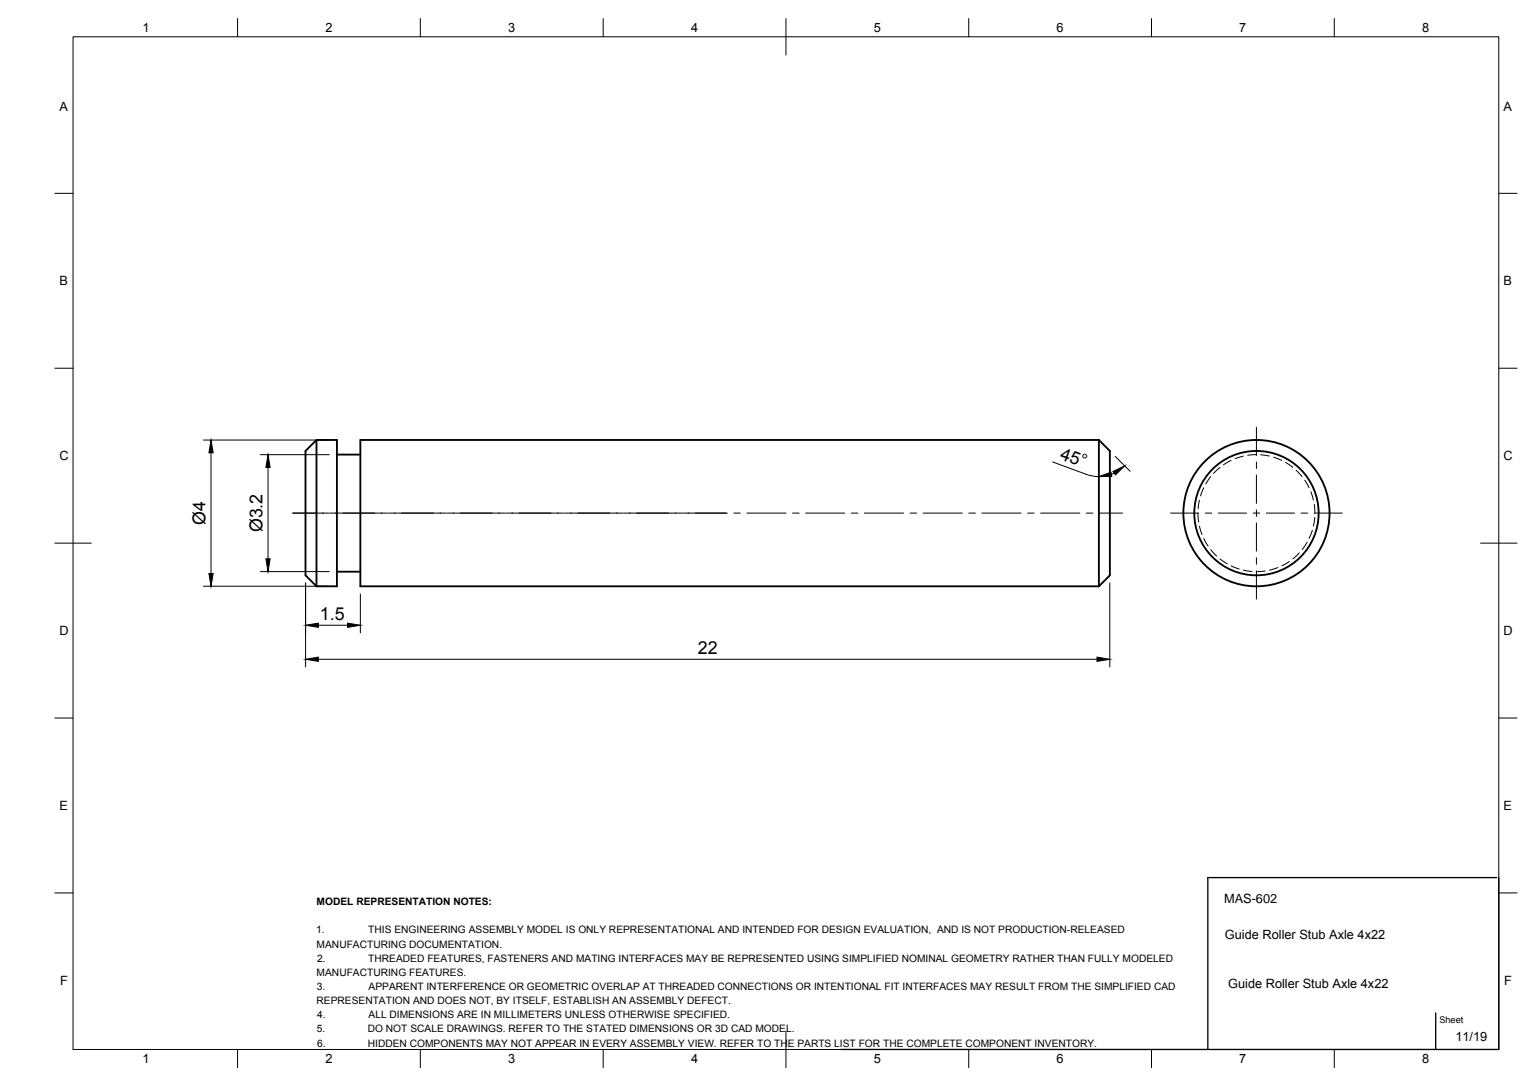
ISO-10303-21;
HEADER;
/* Generated by software containing ST-Developer
 * from STEP Tools, Inc. (www.steptools.com) 
 */

FILE_DESCRIPTION(
/* description */ (''),
/* implementation_level */ '2;1');

FILE_NAME(
/* name */ 'Guide Roller Stub Axle 4x22.step',
/* time_stamp */ '2026-10-15T14:42:47-07:00',
/* author */ (''),
/* organization */ (''),
/* preprocessor_version */ 'ST-DEVELOPER v20.2',
/* originating_system */ 'Autodesk Translation Framework v15.15.0.0',
/* authorisation */ '');

FILE_SCHEMA (('AUTOMOTIVE_DESIGN { 1 0 10303 214 3 1 1 }'));
ENDSEC;

DATA;
#10=MECHANICAL_DESIGN_GEOMETRIC_PRESENTATION_REPRESENTATION('',(#247),#85789);
#187=CONICAL_SURFACE('',#10762,0.185,0.78539816339745);
#188=CONICAL_SURFACE('',#10774,0.185,0.785398163397445);
#211=SHAPE_REPRESENTATION_RELATIONSHIP('SRR','None',#85876,#229);
#229=ADVANCED_BREP_SHAPE_REPRESENTATION('',(#265),#85784);
#247=STYLED_ITEM('',(#85975),#265);
#265=MANIFOLD_SOLID_BREP('Body1',#9894);
#471=FACE_BOUND('',#3409,.T.);
#472=FACE_BOUND('',#3412,.T.);
#1171=PLANE('',#10760);
#1172=PLANE('',#10766);
#1173=PLANE('',#10770);
#1174=PLANE('',#10776);
#1655=LINE('',#77849,#2191);
#1656=LINE('',#77853,#2192);
#1657=LINE('',#77860,#2193);
#1658=LINE('',#77867,#2194);
#1659=LINE('',#77870,#2195);
#2191=VECTOR('',#12747,0.185);
#2192=VECTOR('',#12752,0.2);
#2193=VECTOR('',#12761,0.16);
#2194=VECTOR('',#12770,0.2);
#2195=VECTOR('',#12773,0.185);
#2361=CYLINDRICAL_SURFACE('',#10764,0.2);
#2362=CYLINDRICAL_SURFACE('',#10768,0.16);
#2363=CYLINDRICAL_SURFACE('',#10772,0.2);
#2819=FACE_OUTER_BOUND('',#3405,.T.);
#2820=FACE_OUTER_BOUND('',#3406,.T.);
#2821=FACE_OUTER_BOUND('',#3407,.T.);
#2822=FACE_OUTER_BOUND('',#3408,.T.);
#2823=FACE_OUTER_BOUND('',#3410,.T.);
#2824=FACE_OUTER_BOUND('',#3411,.T.);
#2825=FACE_OUTER_BOUND('',#3413,.T.);
#2826=FACE_OUTER_BOUND('',#3414,.T.);
#2827=FACE_OUTER_BOUND('',#3415,.T.);
#3405=EDGE_LOOP('',(#8863));
#3406=EDGE_LOOP('',(#8864,#8865,#8866,#8867));
#3407=EDGE_LOOP('',(#8868,#8869,#8870,#8871));
#3408=EDGE_LOOP('',(#8872));
#3409=EDGE_LOOP('',(#8873));
#3410=EDGE_LOOP('',(#8874,#8875,#8876,#8877));
#3411=EDGE_LOOP('',(#8878));
#3412=EDGE_LOOP('',(#8879));
#3413=EDGE_LOOP('',(#8880,#8881,#8882,#8883));
#3414=EDGE_LOOP('',(#8884,#8885,#8886,#8887));
#3415=EDGE_LOOP('',(#8888));
#3812=CIRCLE('',#10761,0.17);
#3813=CIRCLE('',#10763,0.2);
#3814=CIRCLE('',#10765,0.2);
#3815=CIRCLE('',#10767,0.16);
#3816=CIRCLE('',#10769,0.16);
#3817=CIRCLE('',#10771,0.2);
#3818=CIRCLE('',#10773,0.2);
#3819=CIRCLE('',#10775,0.17);
#4749=VERTEX_POINT('',#77844);
#4750=VERTEX_POINT('',#77847);
#4751=VERTEX_POINT('',#77851);
#4752=VERTEX_POINT('',#77855);
#4753=VERTEX_POINT('',#77858);
#4754=VERTEX_POINT('',#77862);
#4755=VERTEX_POINT('',#77865);
#4756=VERTEX_POINT('',#77869);
#6159=EDGE_CURVE('',#4749,#4749,#3812,.T.);
#6160=EDGE_CURVE('',#4750,#4750,#3813,.T.);
#6161=EDGE_CURVE('',#4750,#4749,#1655,.T.);
#6162=EDGE_CURVE('',#4751,#4751,#3814,.T.);
#6163=EDGE_CURVE('',#4751,#4750,#1656,.T.);
#6164=EDGE_CURVE('',#4752,#4752,#3815,.T.);
#6165=EDGE_CURVE('',#4753,#4753,#3816,.T.);
#6166=EDGE_CURVE('',#4753,#4752,#1657,.T.);
#6167=EDGE_CURVE('',#4754,#4754,#3817,.T.);
#6168=EDGE_CURVE('',#4755,#4755,#3818,.T.);
#6169=EDGE_CURVE('',#4755,#4754,#1658,.T.);
#6170=EDGE_CURVE('',#4755,#4756,#1659,.T.);
#6171=EDGE_CURVE('',#4756,#4756,#3819,.T.);
#8863=ORIENTED_EDGE('',*,*,#6159,.F.);
#8864=ORIENTED_EDGE('',*,*,#6160,.F.);
#8865=ORIENTED_EDGE('',*,*,#6161,.T.);
#8866=ORIENTED_EDGE('',*,*,#6159,.T.);
#8867=ORIENTED_EDGE('',*,*,#6161,.F.);
#8868=ORIENTED_EDGE('',*,*,#6162,.F.);
#8869=ORIENTED_EDGE('',*,*,#6163,.T.);
#8870=ORIENTED_EDGE('',*,*,#6160,.T.);
#8871=ORIENTED_EDGE('',*,*,#6163,.F.);
#8872=ORIENTED_EDGE('',*,*,#6162,.T.);
#8873=ORIENTED_EDGE('',*,*,#6164,.F.);
#8874=ORIENTED_EDGE('',*,*,#6165,.F.);
#8875=ORIENTED_EDGE('',*,*,#6166,.T.);
#8876=ORIENTED_EDGE('',*,*,#6164,.T.);
#8877=ORIENTED_EDGE('',*,*,#6166,.F.);
#8878=ORIENTED_EDGE('',*,*,#6167,.F.);
#8879=ORIENTED_EDGE('',*,*,#6165,.T.);
#8880=ORIENTED_EDGE('',*,*,#6168,.F.);
#8881=ORIENTED_EDGE('',*,*,#6169,.T.);
#8882=ORIENTED_EDGE('',*,*,#6167,.T.);
#8883=ORIENTED_EDGE('',*,*,#6169,.F.);
#8884=ORIENTED_EDGE('',*,*,#6168,.T.);
#8885=ORIENTED_EDGE('',*,*,#6170,.T.);
#8886=ORIENTED_EDGE('',*,*,#6171,.F.);
#8887=ORIENTED_EDGE('',*,*,#6170,.F.);
#8888=ORIENTED_EDGE('',*,*,#6171,.T.);
#9797=ADVANCED_FACE('',(#2819),#1171,.T.);
#9798=ADVANCED_FACE('',(#2820),#187,.T.);
#9799=ADVANCED_FACE('',(#2821),#2361,.T.);
#9800=ADVANCED_FACE('',(#2822,#471),#1172,.T.);
#9801=ADVANCED_FACE('',(#2823),#2362,.T.);
#9802=ADVANCED_FACE('',(#2824,#472),#1173,.T.);
#9803=ADVANCED_FACE('',(#2825),#2363,.T.);
#9804=ADVANCED_FACE('',(#2826),#188,.T.);
#9805=ADVANCED_FACE('',(#2827),#1174,.T.);
#9894=CLOSED_SHELL('',(#9797,#9798,#9799,#9800,#9801,#9802,#9803,#9804,
#9805));
#10759=AXIS2_PLACEMENT_3D('',#77842,#12737,#12738);
#10760=AXIS2_PLACEMENT_3D('',#77843,#12739,#12740);
#10761=AXIS2_PLACEMENT_3D('',#77845,#12741,#12742);
#10762=AXIS2_PLACEMENT_3D('',#77846,#12743,#12744);
#10763=AXIS2_PLACEMENT_3D('',#77848,#12745,#12746);
#10764=AXIS2_PLACEMENT_3D('',#77850,#12748,#12749);
#10765=AXIS2_PLACEMENT_3D('',#77852,#12750,#12751);
#10766=AXIS2_PLACEMENT_3D('',#77854,#12753,#12754);
#10767=AXIS2_PLACEMENT_3D('',#77856,#12755,#12756);
#10768=AXIS2_PLACEMENT_3D('',#77857,#12757,#12758);
#10769=AXIS2_PLACEMENT_3D('',#77859,#12759,#12760);
#10770=AXIS2_PLACEMENT_3D('',#77861,#12762,#12763);
#10771=AXIS2_PLACEMENT_3D('',#77863,#12764,#12765);
#10772=AXIS2_PLACEMENT_3D('',#77864,#12766,#12767);
#10773=AXIS2_PLACEMENT_3D('',#77866,#12768,#12769);
#10774=AXIS2_PLACEMENT_3D('',#77868,#12771,#12772);
#10775=AXIS2_PLACEMENT_3D('',#77871,#12774,#12775);
#10776=AXIS2_PLACEMENT_3D('',#77872,#12776,#12777);
#12737=DIRECTION('axis',(0.,0.,1.));
#12738=DIRECTION('refdir',(1.,0.,0.));
#12739=DIRECTION('center_axis',(-1.,0.,0.));
#12740=DIRECTION('ref_axis',(0.,0.,1.));
#12741=DIRECTION('center_axis',(1.,0.,0.));
#12742=DIRECTION('ref_axis',(0.,0.,-1.));
#12743=DIRECTION('center_axis',(1.,0.,0.));
#12744=DIRECTION('ref_axis',(0.,1.,0.));
#12745=DIRECTION('center_axis',(1.,0.,0.));
#12746=DIRECTION('ref_axis',(0.,0.,-1.));
#12747=DIRECTION('',(-0.707106781186546,0.707106781186549,8.65956056235495E-17));
#12748=DIRECTION('center_axis',(1.,0.,0.));
#12749=DIRECTION('ref_axis',(0.,1.,0.));
#12750=DIRECTION('center_axis',(1.,0.,0.));
#12751=DIRECTION('ref_axis',(0.,0.,-1.));
#12752=DIRECTION('',(-1.,0.,0.));
#12753=DIRECTION('center_axis',(1.,0.,0.));
#12754=DIRECTION('ref_axis',(0.,0.,-1.));
#12755=DIRECTION('center_axis',(1.,0.,0.));
#12756=DIRECTION('ref_axis',(0.,0.,-1.));
#12757=DIRECTION('center_axis',(1.,0.,0.));
#12758=DIRECTION('ref_axis',(0.,1.,0.));
#12759=DIRECTION('center_axis',(1.,0.,0.));
#12760=DIRECTION('ref_axis',(0.,0.,-1.));
#12761=DIRECTION('',(-1.,0.,0.));
#12762=DIRECTION('center_axis',(-1.,0.,0.));
#12763=DIRECTION('ref_axis',(0.,0.,1.));
#12764=DIRECTION('center_axis',(1.,0.,0.));
#12765=DIRECTION('ref_axis',(0.,0.,-1.));
#12766=DIRECTION('center_axis',(1.,0.,0.));
#12767=DIRECTION('ref_axis',(0.,1.,0.));
#12768=DIRECTION('center_axis',(1.,0.,0.));
#12769=DIRECTION('ref_axis',(0.,0.,-1.));
#12770=DIRECTION('',(-1.,0.,0.));
#12771=DIRECTION('center_axis',(-1.,0.,0.));
#12772=DIRECTION('ref_axis',(0.,1.,0.));
#12773=DIRECTION('',(0.70710678118655,0.707106781186545,-8.6595605623549E-17));
#12774=DIRECTION('center_axis',(1.,0.,0.));
#12775=DIRECTION('ref_axis',(0.,0.,-1.));
#12776=DIRECTION('center_axis',(1.,0.,0.));
#12777=DIRECTION('ref_axis',(0.,0.,-1.));
#77842=CARTESIAN_POINT('',(0.,0.,0.));
#77843=CARTESIAN_POINT('Origin',(0.55,0.17,0.));
#77844=CARTESIAN_POINT('',(0.55,-0.17,-2.0818995585505E-17));
#77845=CARTESIAN_POINT('Origin',(0.55,0.,0.));
#77846=CARTESIAN_POINT('Origin',(0.565,0.,0.));
#77847=CARTESIAN_POINT('',(0.58,-0.2,-2.44929359829471E-17));
#77848=CARTESIAN_POINT('Origin',(0.58,0.,0.));
#77849=CARTESIAN_POINT('',(0.565,-0.185,-2.2655965784226E-17));
#77850=CARTESIAN_POINT('Origin',(1.59,0.,0.));
#77851=CARTESIAN_POINT('',(2.6,-0.2,-2.44929359829471E-17));
#77852=CARTESIAN_POINT('Origin',(2.6,0.,0.));
#77853=CARTESIAN_POINT('',(1.59,-0.2,-2.44929359829471E-17));
#77854=CARTESIAN_POINT('Origin',(2.6,0.16,0.));
#77855=CARTESIAN_POINT('',(2.6,-0.16,-1.95943487863577E-17));
#77856=CARTESIAN_POINT('Origin',(2.6,0.,0.));
#77857=CARTESIAN_POINT('Origin',(2.632,0.,0.));
#77858=CARTESIAN_POINT('',(2.664,-0.16,-1.95943487863577E-17));
#77859=CARTESIAN_POINT('Origin',(2.664,0.,0.));
#77860=CARTESIAN_POINT('',(2.632,-0.16,-1.95943487863577E-17));
#77861=CARTESIAN_POINT('Origin',(2.664,0.2,0.));
#77862=CARTESIAN_POINT('',(2.664,-0.2,-2.44929359829471E-17));
#77863=CARTESIAN_POINT('Origin',(2.664,0.,0.));
#77864=CARTESIAN_POINT('Origin',(2.692,0.,0.));
#77865=CARTESIAN_POINT('',(2.72,-0.2,-2.44929359829471E-17));
#77866=CARTESIAN_POINT('Origin',(2.72,0.,0.));
#77867=CARTESIAN_POINT('',(2.692,-0.2,-2.44929359829471E-17));
#77868=CARTESIAN_POINT('Origin',(2.735,0.,0.));
#77869=CARTESIAN_POINT('',(2.75,-0.17,-2.0818995585505E-17));
#77870=CARTESIAN_POINT('',(2.735,-0.185,2.2655965784226E-17));
#77871=CARTESIAN_POINT('Origin',(2.75,0.,0.));
#77872=CARTESIAN_POINT('Origin',(2.75,0.,0.));
#85764=UNCERTAINTY_MEASURE_WITH_UNIT(LENGTH_MEASURE(0.001),#85790,
'DISTANCE_ACCURACY_VALUE',
'Maximum model space distance between geometric entities at asserted c
onnectivities');
#85769=UNCERTAINTY_MEASURE_WITH_UNIT(LENGTH_MEASURE(0.001),#85790,
'DISTANCE_ACCURACY_VALUE',
'Maximum model space distance between geometric entities at asserted c
onnectivities');
#85784=(
GEOMETRIC_REPRESENTATION_CONTEXT(3)
GLOBAL_UNCERTAINTY_ASSIGNED_CONTEXT((#85764))
GLOBAL_UNIT_ASSIGNED_CONTEXT((#85790,#85792,#85793))
REPRESENTATION_CONTEXT('','3D')
);
#85789=(
GEOMETRIC_REPRESENTATION_CONTEXT(3)
GLOBAL_UNCERTAINTY_ASSIGNED_CONTEXT((#85769))
GLOBAL_UNIT_ASSIGNED_CONTEXT((#85790,#85792,#85793))
REPRESENTATION_CONTEXT('','3D')
);
#85790=(
LENGTH_UNIT()
NAMED_UNIT(*)
SI_UNIT(.CENTI.,.METRE.)
);
#85792=(
NAMED_UNIT(*)
PLANE_ANGLE_UNIT()
SI_UNIT($,.RADIAN.)
);
#85793=(
NAMED_UNIT(*)
SI_UNIT($,.STERADIAN.)
SOLID_ANGLE_UNIT()
);
#85808=SHAPE_DEFINITION_REPRESENTATION(#85827,#85876);
#85827=PRODUCT_DEFINITION_SHAPE('',$,#85896);
#85876=SHAPE_REPRESENTATION('',(#10759),#85784);
#85881=PRODUCT_DEFINITION_CONTEXT('part definition',#85940,'design');
#85896=PRODUCT_DEFINITION('Guide Roller Stub Axle 4x22',
'Guide Roller Stub Axle 4x22',#85915,#85881);
#85915=PRODUCT_DEFINITION_FORMATION('',$,#85956);
#85940=APPLICATION_CONTEXT(
'Core Data for Automotive Mechanical Design Process');
#85941=PRODUCT_CONTEXT('part definition',#85940,'mechanical');
#85956=PRODUCT('Guide Roller Stub Axle 4x22',
'Guide Roller Stub Axle 4x22',$,(#85941));
#85975=PRESENTATION_STYLE_ASSIGNMENT((#85993));
#85993=SURFACE_STYLE_USAGE(.BOTH.,#86011);
#86011=SURFACE_SIDE_STYLE('',(#86029));
#86029=SURFACE_STYLE_FILL_AREA(#86047);
#86047=FILL_AREA_STYLE('Opaque(214,217,222)',(#86065));
#86065=FILL_AREA_STYLE_COLOUR('Opaque(214,217,222)',#86083);
#86083=COLOUR_RGB('Opaque(214,217,222)', 0.31764706, 0.68627451, 0.89019608);
ENDSEC;
END-ISO-10303-21;
